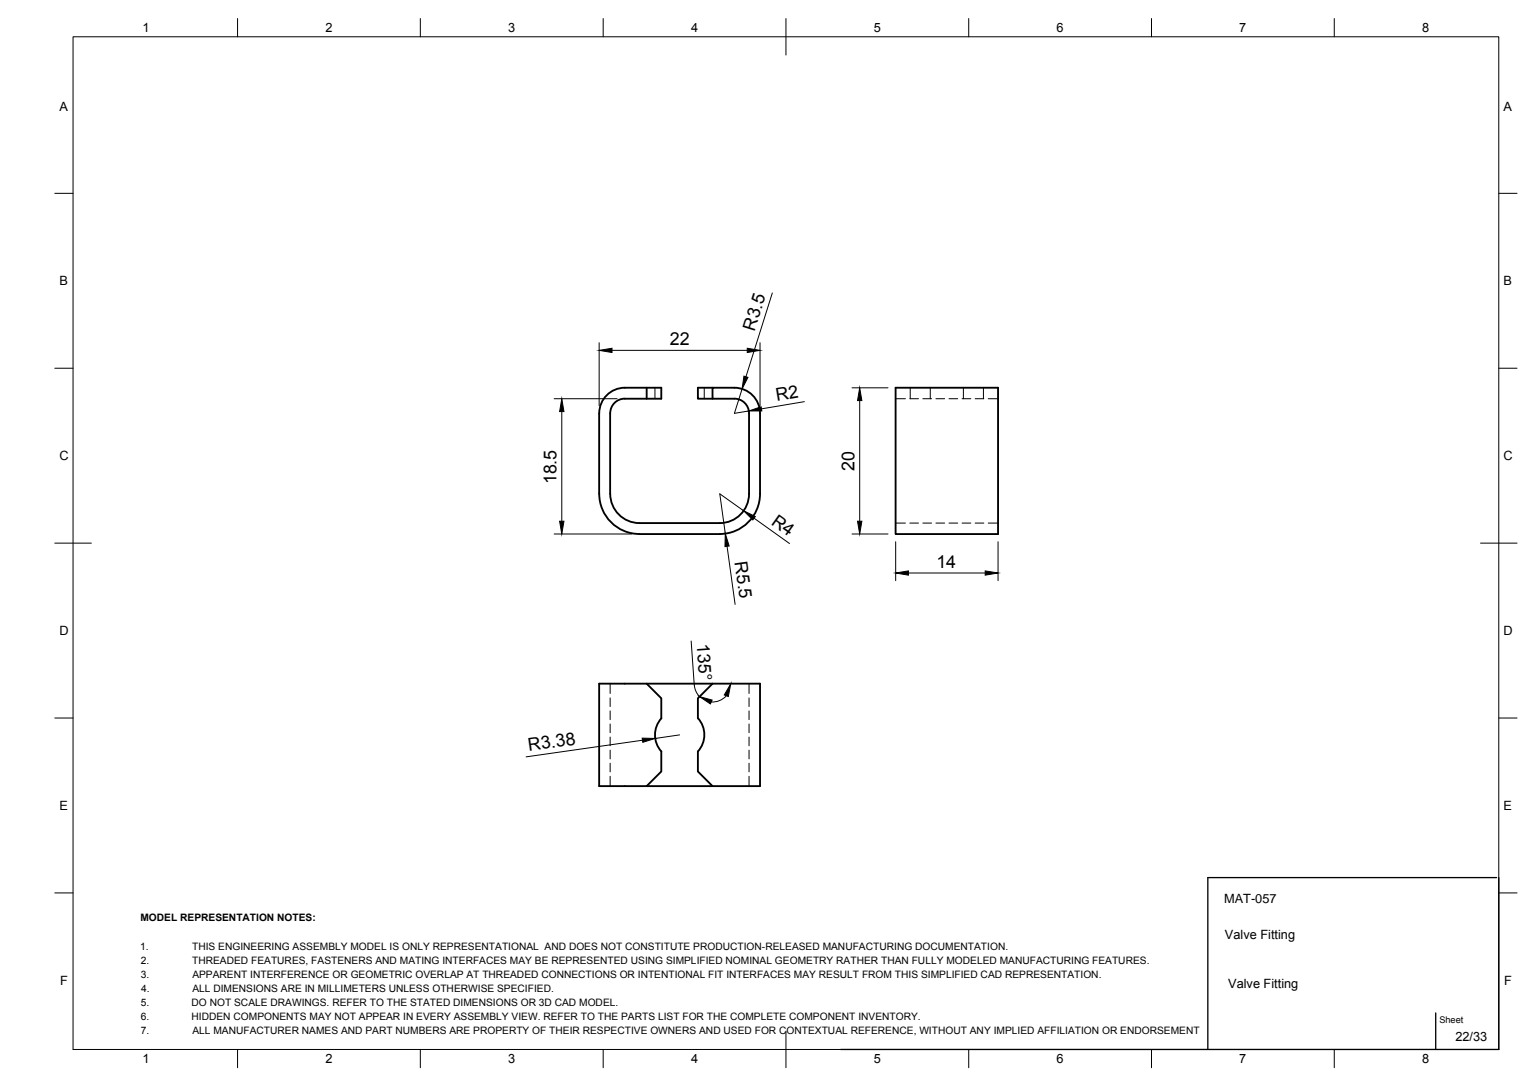
ISO-10303-21;
HEADER;
/* Generated by software containing ST-Developer
 * from STEP Tools, Inc. (www.steptools.com) 
 */

FILE_DESCRIPTION(
/* description */ ('STEP AP214', 'CAx-IF Rec.Pracs.---Representation and Presentation of Product Manufa
cturing Information (PMI)---4.0---2014-10-13'),
/* implementation_level */ '2;1');

FILE_NAME(
/* name */ 'Valve Fitting.step',
/* time_stamp */ '2026-10-28T23:34:22+01:00',
/* author */ (''),
/* organization */ (''),
/* preprocessor_version */ 'ST-DEVELOPER v20.2',
/* originating_system */ 'Autodesk Translation Framework v15.17.0.0',
/* authorisation */ '');

FILE_SCHEMA (('AP242_MANAGED_MODEL_BASED_3D_ENGINEERING_MIM_LF { 1 0 10303 442 2 1 4 }'));
ENDSEC;

DATA;
#10=MECHANICAL_DESIGN_GEOMETRIC_PRESENTATION_REPRESENTATION('',(#263),#27807);
#217=SHAPE_REPRESENTATION_RELATIONSHIP('SRR','None',#27914,#239);
#239=ADVANCED_BREP_SHAPE_REPRESENTATION('',(#292),#27794);
#263=STYLED_ITEM('',(#28070),#292);
#292=MANIFOLD_SOLID_BREP('Body1',#12039);
#645=PLANE('',#13213);
#646=PLANE('',#13215);
#647=PLANE('',#13217);
#648=PLANE('',#13226);
#649=PLANE('',#13236);
#650=PLANE('',#13238);
#651=PLANE('',#13240);
#652=PLANE('',#13242);
#653=PLANE('',#13245);
#654=PLANE('',#13247);
#655=PLANE('',#13249);
#656=PLANE('',#13251);
#657=PLANE('',#13253);
#658=PLANE('',#13255);
#659=PLANE('',#13256);
#660=PLANE('',#13258);
#661=PLANE('',#13259);
#662=PLANE('',#13260);
#663=PLANE('',#13261);
#664=PLANE('',#13262);
#1141=CYLINDRICAL_SURFACE('',#13235,3.49999999999998);
#1142=CYLINDRICAL_SURFACE('',#13237,5.50000000000002);
#1143=CYLINDRICAL_SURFACE('',#13239,5.50000000000002);
#1144=CYLINDRICAL_SURFACE('',#13241,3.49999999999998);
#1145=CYLINDRICAL_SURFACE('',#13244,1.99999999999999);
#1146=CYLINDRICAL_SURFACE('',#13246,3.99999999999998);
#1147=CYLINDRICAL_SURFACE('',#13248,3.99999999999998);
#1148=CYLINDRICAL_SURFACE('',#13250,1.99999999999999);
#1149=CYLINDRICAL_SURFACE('',#13254,3.37500000000002);
#1150=CYLINDRICAL_SURFACE('',#13257,3.37500000000002);
#1676=FACE_OUTER_BOUND('',#2452,.T.);
#1677=FACE_OUTER_BOUND('',#2453,.T.);
#1678=FACE_OUTER_BOUND('',#2454,.T.);
#1679=FACE_OUTER_BOUND('',#2455,.T.);
#1680=FACE_OUTER_BOUND('',#2456,.T.);
#1681=FACE_OUTER_BOUND('',#2457,.T.);
#1682=FACE_OUTER_BOUND('',#2458,.T.);
#1683=FACE_OUTER_BOUND('',#2459,.T.);
#1684=FACE_OUTER_BOUND('',#2460,.T.);
#1685=FACE_OUTER_BOUND('',#2461,.T.);
#1686=FACE_OUTER_BOUND('',#2462,.T.);
#1687=FACE_OUTER_BOUND('',#2463,.T.);
#1688=FACE_OUTER_BOUND('',#2464,.T.);
#1689=FACE_OUTER_BOUND('',#2465,.T.);
#1690=FACE_OUTER_BOUND('',#2466,.T.);
#1691=FACE_OUTER_BOUND('',#2467,.T.);
#1692=FACE_OUTER_BOUND('',#2468,.T.);
#1693=FACE_OUTER_BOUND('',#2469,.T.);
#1694=FACE_OUTER_BOUND('',#2470,.T.);
#1695=FACE_OUTER_BOUND('',#2471,.T.);
#1696=FACE_OUTER_BOUND('',#2472,.T.);
#1697=FACE_OUTER_BOUND('',#2473,.T.);
#1698=FACE_OUTER_BOUND('',#2474,.T.);
#1699=FACE_OUTER_BOUND('',#2475,.T.);
#1700=FACE_OUTER_BOUND('',#2476,.T.);
#1701=FACE_OUTER_BOUND('',#2477,.T.);
#1702=FACE_OUTER_BOUND('',#2478,.T.);
#1703=FACE_OUTER_BOUND('',#2479,.T.);
#1704=FACE_OUTER_BOUND('',#2480,.T.);
#1705=FACE_OUTER_BOUND('',#2481,.T.);
#2452=EDGE_LOOP('',(#9995,#9996,#9997,#9998,#9999,#10000,#10001,#10002));
#2453=EDGE_LOOP('',(#10003,#10004,#10005,#10006,#10007,#10008,#10009,#10010));
#2454=EDGE_LOOP('',(#10011,#10012,#10013,#10014,#10015,#10016,#10017,#10018,
#10019,#10020,#10021,#10022,#10023,#10024,#10025,#10026,#10027,#10028,#10029,
#10030));
#2455=EDGE_LOOP('',(#10031,#10032,#10033,#10034,#10035,#10036,#10037,#10038,
#10039,#10040,#10041,#10042,#10043,#10044,#10045,#10046,#10047,#10048,#10049,
#10050));
#2456=EDGE_LOOP('',(#10051,#10052,#10053,#10054));
#2457=EDGE_LOOP('',(#10055,#10056,#10057,#10058));
#2458=EDGE_LOOP('',(#10059,#10060,#10061,#10062));
#2459=EDGE_LOOP('',(#10063,#10064,#10065,#10066));
#2460=EDGE_LOOP('',(#10067,#10068,#10069,#10070));
#2461=EDGE_LOOP('',(#10071,#10072,#10073,#10074));
#2462=EDGE_LOOP('',(#10075,#10076,#10077,#10078));
#2463=EDGE_LOOP('',(#10079,#10080,#10081,#10082,#10083,#10084,#10085,#10086));
#2464=EDGE_LOOP('',(#10087,#10088,#10089,#10090));
#2465=EDGE_LOOP('',(#10091,#10092,#10093,#10094));
#2466=EDGE_LOOP('',(#10095,#10096,#10097,#10098));
#2467=EDGE_LOOP('',(#10099,#10100,#10101,#10102));
#2468=EDGE_LOOP('',(#10103,#10104,#10105,#10106));
#2469=EDGE_LOOP('',(#10107,#10108,#10109,#10110));
#2470=EDGE_LOOP('',(#10111,#10112,#10113,#10114));
#2471=EDGE_LOOP('',(#10115,#10116,#10117,#10118,#10119,#10120,#10121,#10122));
#2472=EDGE_LOOP('',(#10123,#10124,#10125,#10126));
#2473=EDGE_LOOP('',(#10127,#10128,#10129,#10130));
#2474=EDGE_LOOP('',(#10131,#10132,#10133,#10134));
#2475=EDGE_LOOP('',(#10135,#10136,#10137,#10138));
#2476=EDGE_LOOP('',(#10139,#10140,#10141,#10142));
#2477=EDGE_LOOP('',(#10143,#10144,#10145,#10146));
#2478=EDGE_LOOP('',(#10147,#10148,#10149,#10150));
#2479=EDGE_LOOP('',(#10151,#10152,#10153,#10154));
#2480=EDGE_LOOP('',(#10155,#10156,#10157,#10158));
#2481=EDGE_LOOP('',(#10159,#10160,#10161,#10162));
#3280=LINE('',#21304,#4100);
#3281=LINE('',#21306,#4101);
#3282=LINE('',#21308,#4102);
#3283=LINE('',#21310,#4103);
#3284=LINE('',#21312,#4104);
#3285=LINE('',#21314,#4105);
#3286=LINE('',#21316,#4106);
#3287=LINE('',#21321,#4107);
#3288=LINE('',#21323,#4108);
#3289=LINE('',#21325,#4109);
#3290=LINE('',#21329,#4110);
#3291=LINE('',#21331,#4111);
#3292=LINE('',#21333,#4112);
#3293=LINE('',#21334,#4113);
#3294=LINE('',#21336,#4114);
#3295=LINE('',#21340,#4115);
#3296=LINE('',#21344,#4116);
#3297=LINE('',#21348,#4117);
#3298=LINE('',#21352,#4118);
#3299=LINE('',#21354,#4119);
#3300=LINE('',#21356,#4120);
#3301=LINE('',#21360,#4121);
#3302=LINE('',#21364,#4122);
#3303=LINE('',#21368,#4123);
#3304=LINE('',#21373,#4124);
#3305=LINE('',#21375,#4125);
#3306=LINE('',#21377,#4126);
#3307=LINE('',#21381,#4127);
#3308=LINE('',#21385,#4128);
#3309=LINE('',#21389,#4129);
#3310=LINE('',#21391,#4130);
#3311=LINE('',#21395,#4131);
#3312=LINE('',#21399,#4132);
#3313=LINE('',#21403,#4133);
#3314=LINE('',#21406,#4134);
#3315=LINE('',#21408,#4135);
#3316=LINE('',#21410,#4136);
#3317=LINE('',#21412,#4137);
#3318=LINE('',#21414,#4138);
#3319=LINE('',#21416,#4139);
#3320=LINE('',#21418,#4140);
#3321=LINE('',#21421,#4141);
#3322=LINE('',#21423,#4142);
#3323=LINE('',#21427,#4143);
#3324=LINE('',#21428,#4144);
#3325=LINE('',#21430,#4145);
#3326=LINE('',#21432,#4146);
#3327=LINE('',#21434,#4147);
#3328=LINE('',#21436,#4148);
#3329=LINE('',#21438,#4149);
#3330=LINE('',#21440,#4150);
#3331=LINE('',#21442,#4151);
#3332=LINE('',#21446,#4152);
#3333=LINE('',#21447,#4153);
#3334=LINE('',#21449,#4154);
#3335=LINE('',#21451,#4155);
#3336=LINE('',#21454,#4156);
#3337=LINE('',#21455,#4157);
#3338=LINE('',#21457,#4158);
#3339=LINE('',#21459,#4159);
#3340=LINE('',#21461,#4160);
#3341=LINE('',#21462,#4161);
#3342=LINE('',#21464,#4162);
#3343=LINE('',#21466,#4163);
#4100=VECTOR('',#16090,1000.);
#4101=VECTOR('',#16091,1000.);
#4102=VECTOR('',#16092,1000.);
#4103=VECTOR('',#16093,1000.);
#4104=VECTOR('',#16094,1000.);
#4105=VECTOR('',#16095,1000.);
#4106=VECTOR('',#16096,1000.);
#4107=VECTOR('',#16101,1000.);
#4108=VECTOR('',#16102,1000.);
#4109=VECTOR('',#16103,1000.);
#4110=VECTOR('',#16106,1000.);
#4111=VECTOR('',#16107,1000.);
#4112=VECTOR('',#16108,1000.);
#4113=VECTOR('',#16109,1000.);
#4114=VECTOR('',#16112,1000.);
#4115=VECTOR('',#16115,1000.);
#4116=VECTOR('',#16118,1000.);
#4117=VECTOR('',#16121,1000.);
#4118=VECTOR('',#16124,1000.);
#4119=VECTOR('',#16125,1000.);
#4120=VECTOR('',#16126,1000.);
#4121=VECTOR('',#16129,1000.);
#4122=VECTOR('',#16132,1000.);
#4123=VECTOR('',#16135,1000.);
#4124=VECTOR('',#16140,1000.);
#4125=VECTOR('',#16141,1000.);
#4126=VECTOR('',#16142,1000.);
#4127=VECTOR('',#16145,1000.);
#4128=VECTOR('',#16148,1000.);
#4129=VECTOR('',#16151,1000.);
#4130=VECTOR('',#16154,1000.);
#4131=VECTOR('',#16157,1000.);
#4132=VECTOR('',#16160,1000.);
#4133=VECTOR('',#16163,1000.);
#4134=VECTOR('',#16168,1000.);
#4135=VECTOR('',#16171,1000.);
#4136=VECTOR('',#16174,1000.);
#4137=VECTOR('',#16177,1000.);
#4138=VECTOR('',#16180,1000.);
#4139=VECTOR('',#16183,1000.);
#4140=VECTOR('',#16186,1000.);
#4141=VECTOR('',#16189,1000.);
#4142=VECTOR('',#16190,1000.);
#4143=VECTOR('',#16193,1000.);
#4144=VECTOR('',#16194,1000.);
#4145=VECTOR('',#16197,1000.);
#4146=VECTOR('',#16200,1000.);
#4147=VECTOR('',#16203,1000.);
#4148=VECTOR('',#16206,1000.);
#4149=VECTOR('',#16209,1000.);
#4150=VECTOR('',#16212,1000.);
#4151=VECTOR('',#16215,1000.);
#4152=VECTOR('',#16218,1000.);
#4153=VECTOR('',#16219,1000.);
#4154=VECTOR('',#16220,1000.);
#4155=VECTOR('',#16221,1000.);
#4156=VECTOR('',#16226,1000.);
#4157=VECTOR('',#16227,1000.);
#4158=VECTOR('',#16230,1000.);
#4159=VECTOR('',#16233,1000.);
#4160=VECTOR('',#16236,1000.);
#4161=VECTOR('',#16237,1000.);
#4162=VECTOR('',#16240,1000.);
#4163=VECTOR('',#16243,1000.);
#4813=CIRCLE('',#13214,3.37500000000002);
#4814=CIRCLE('',#13216,3.37500000000002);
#4815=CIRCLE('',#13218,3.49999999999998);
#4816=CIRCLE('',#13219,5.50000000000002);
#4817=CIRCLE('',#13220,5.50000000000002);
#4818=CIRCLE('',#13221,3.49999999999998);
#4819=CIRCLE('',#13222,1.99999999999999);
#4820=CIRCLE('',#13223,3.99999999999998);
#4821=CIRCLE('',#13224,3.99999999999998);
#4822=CIRCLE('',#13225,1.99999999999999);
#4823=CIRCLE('',#13227,3.49999999999998);
#4824=CIRCLE('',#13228,5.50000000000002);
#4825=CIRCLE('',#13229,5.50000000000002);
#4826=CIRCLE('',#13230,3.49999999999998);
#4827=CIRCLE('',#13231,1.99999999999999);
#4828=CIRCLE('',#13232,3.99999999999998);
#4829=CIRCLE('',#13233,3.99999999999998);
#4830=CIRCLE('',#13234,1.99999999999999);
#4831=CIRCLE('',#13243,3.37500000000002);
#4832=CIRCLE('',#13252,3.37500000000002);
#5725=VERTEX_POINT('',#21302);
#5726=VERTEX_POINT('',#21303);
#5727=VERTEX_POINT('',#21305);
#5728=VERTEX_POINT('',#21307);
#5729=VERTEX_POINT('',#21309);
#5730=VERTEX_POINT('',#21311);
#5731=VERTEX_POINT('',#21313);
#5732=VERTEX_POINT('',#21315);
#5733=VERTEX_POINT('',#21319);
#5734=VERTEX_POINT('',#21320);
#5735=VERTEX_POINT('',#21322);
#5736=VERTEX_POINT('',#21324);
#5737=VERTEX_POINT('',#21326);
#5738=VERTEX_POINT('',#21328);
#5739=VERTEX_POINT('',#21330);
#5740=VERTEX_POINT('',#21332);
#5741=VERTEX_POINT('',#21337);
#5742=VERTEX_POINT('',#21339);
#5743=VERTEX_POINT('',#21341);
#5744=VERTEX_POINT('',#21343);
#5745=VERTEX_POINT('',#21345);
#5746=VERTEX_POINT('',#21347);
#5747=VERTEX_POINT('',#21349);
#5748=VERTEX_POINT('',#21351);
#5749=VERTEX_POINT('',#21353);
#5750=VERTEX_POINT('',#21355);
#5751=VERTEX_POINT('',#21357);
#5752=VERTEX_POINT('',#21359);
#5753=VERTEX_POINT('',#21361);
#5754=VERTEX_POINT('',#21363);
#5755=VERTEX_POINT('',#21365);
#5756=VERTEX_POINT('',#21367);
#5757=VERTEX_POINT('',#21371);
#5758=VERTEX_POINT('',#21372);
#5759=VERTEX_POINT('',#21374);
#5760=VERTEX_POINT('',#21376);
#5761=VERTEX_POINT('',#21378);
#5762=VERTEX_POINT('',#21380);
#5763=VERTEX_POINT('',#21382);
#5764=VERTEX_POINT('',#21384);
#5765=VERTEX_POINT('',#21386);
#5766=VERTEX_POINT('',#21388);
#5767=VERTEX_POINT('',#21392);
#5768=VERTEX_POINT('',#21394);
#5769=VERTEX_POINT('',#21396);
#5770=VERTEX_POINT('',#21398);
#5771=VERTEX_POINT('',#21400);
#5772=VERTEX_POINT('',#21402);
#5773=VERTEX_POINT('',#21420);
#5774=VERTEX_POINT('',#21422);
#5775=VERTEX_POINT('',#21424);
#5776=VERTEX_POINT('',#21426);
#5777=VERTEX_POINT('',#21444);
#5778=VERTEX_POINT('',#21445);
#5779=VERTEX_POINT('',#21448);
#5780=VERTEX_POINT('',#21450);
#7210=EDGE_CURVE('',#5725,#5726,#3280,.T.);
#7211=EDGE_CURVE('',#5725,#5727,#3281,.T.);
#7212=EDGE_CURVE('',#5727,#5728,#3282,.T.);
#7213=EDGE_CURVE('',#5729,#5728,#3283,.T.);
#7214=EDGE_CURVE('',#5730,#5729,#3284,.T.);
#7215=EDGE_CURVE('',#5730,#5731,#3285,.T.);
#7216=EDGE_CURVE('',#5732,#5731,#3286,.T.);
#7217=EDGE_CURVE('',#5726,#5732,#4813,.T.);
#7218=EDGE_CURVE('',#5733,#5734,#3287,.T.);
#7219=EDGE_CURVE('',#5733,#5735,#3288,.T.);
#7220=EDGE_CURVE('',#5736,#5735,#3289,.T.);
#7221=EDGE_CURVE('',#5737,#5736,#4814,.T.);
#7222=EDGE_CURVE('',#5738,#5737,#3290,.T.);
#7223=EDGE_CURVE('',#5738,#5739,#3291,.T.);
#7224=EDGE_CURVE('',#5739,#5740,#3292,.T.);
#7225=EDGE_CURVE('',#5740,#5734,#3293,.T.);
#7226=EDGE_CURVE('',#5739,#5730,#3294,.T.);
#7227=EDGE_CURVE('',#5729,#5741,#4815,.T.);
#7228=EDGE_CURVE('',#5741,#5742,#3295,.T.);
#7229=EDGE_CURVE('',#5742,#5743,#4816,.T.);
#7230=EDGE_CURVE('',#5743,#5744,#3296,.T.);
#7231=EDGE_CURVE('',#5744,#5745,#4817,.T.);
#7232=EDGE_CURVE('',#5745,#5746,#3297,.T.);
#7233=EDGE_CURVE('',#5746,#5747,#4818,.T.);
#7234=EDGE_CURVE('',#5747,#5748,#3298,.T.);
#7235=EDGE_CURVE('',#5748,#5749,#3299,.T.);
#7236=EDGE_CURVE('',#5750,#5749,#3300,.T.);
#7237=EDGE_CURVE('',#5751,#5750,#4819,.T.);
#7238=EDGE_CURVE('',#5752,#5751,#3301,.T.);
#7239=EDGE_CURVE('',#5753,#5752,#4820,.T.);
#7240=EDGE_CURVE('',#5754,#5753,#3302,.T.);
#7241=EDGE_CURVE('',#5755,#5754,#4821,.T.);
#7242=EDGE_CURVE('',#5756,#5755,#3303,.T.);
#7243=EDGE_CURVE('',#5740,#5756,#4822,.T.);
#7244=EDGE_CURVE('',#5757,#5758,#3304,.T.);
#7245=EDGE_CURVE('',#5758,#5759,#3305,.T.);
#7246=EDGE_CURVE('',#5760,#5759,#3306,.T.);
#7247=EDGE_CURVE('',#5761,#5760,#4823,.T.);
#7248=EDGE_CURVE('',#5762,#5761,#3307,.T.);
#7249=EDGE_CURVE('',#5763,#5762,#4824,.T.);
#7250=EDGE_CURVE('',#5764,#5763,#3308,.T.);
#7251=EDGE_CURVE('',#5765,#5764,#4825,.T.);
#7252=EDGE_CURVE('',#5766,#5765,#3309,.T.);
#7253=EDGE_CURVE('',#5728,#5766,#4826,.T.);
#7254=EDGE_CURVE('',#5727,#5733,#3310,.T.);
#7255=EDGE_CURVE('',#5734,#5767,#4827,.T.);
#7256=EDGE_CURVE('',#5767,#5768,#3311,.T.);
#7257=EDGE_CURVE('',#5768,#5769,#4828,.T.);
#7258=EDGE_CURVE('',#5769,#5770,#3312,.T.);
#7259=EDGE_CURVE('',#5770,#5771,#4829,.T.);
#7260=EDGE_CURVE('',#5771,#5772,#3313,.T.);
#7261=EDGE_CURVE('',#5772,#5757,#4830,.T.);
#7262=EDGE_CURVE('',#5741,#5766,#3314,.T.);
#7263=EDGE_CURVE('',#5742,#5765,#3315,.T.);
#7264=EDGE_CURVE('',#5743,#5764,#3316,.T.);
#7265=EDGE_CURVE('',#5744,#5763,#3317,.T.);
#7266=EDGE_CURVE('',#5745,#5762,#3318,.T.);
#7267=EDGE_CURVE('',#5746,#5761,#3319,.T.);
#7268=EDGE_CURVE('',#5747,#5760,#3320,.T.);
#7269=EDGE_CURVE('',#5759,#5773,#3321,.T.);
#7270=EDGE_CURVE('',#5774,#5773,#3322,.T.);
#7271=EDGE_CURVE('',#5775,#5774,#4831,.T.);
#7272=EDGE_CURVE('',#5776,#5775,#3323,.T.);
#7273=EDGE_CURVE('',#5776,#5748,#3324,.T.);
#7274=EDGE_CURVE('',#5756,#5767,#3325,.T.);
#7275=EDGE_CURVE('',#5755,#5768,#3326,.T.);
#7276=EDGE_CURVE('',#5754,#5769,#3327,.T.);
#7277=EDGE_CURVE('',#5753,#5770,#3328,.T.);
#7278=EDGE_CURVE('',#5752,#5771,#3329,.T.);
#7279=EDGE_CURVE('',#5751,#5772,#3330,.T.);
#7280=EDGE_CURVE('',#5750,#5757,#3331,.T.);
#7281=EDGE_CURVE('',#5777,#5778,#3332,.T.);
#7282=EDGE_CURVE('',#5777,#5758,#3333,.T.);
#7283=EDGE_CURVE('',#5749,#5779,#3334,.T.);
#7284=EDGE_CURVE('',#5780,#5779,#3335,.T.);
#7285=EDGE_CURVE('',#5778,#5780,#4832,.T.);
#7286=EDGE_CURVE('',#5779,#5776,#3336,.T.);
#7287=EDGE_CURVE('',#5780,#5775,#3337,.T.);
#7288=EDGE_CURVE('',#5778,#5774,#3338,.T.);
#7289=EDGE_CURVE('',#5773,#5777,#3339,.T.);
#7290=EDGE_CURVE('',#5731,#5738,#3340,.T.);
#7291=EDGE_CURVE('',#5737,#5732,#3341,.T.);
#7292=EDGE_CURVE('',#5736,#5726,#3342,.T.);
#7293=EDGE_CURVE('',#5735,#5725,#3343,.T.);
#9995=ORIENTED_EDGE('',*,*,#7210,.F.);
#9996=ORIENTED_EDGE('',*,*,#7211,.T.);
#9997=ORIENTED_EDGE('',*,*,#7212,.T.);
#9998=ORIENTED_EDGE('',*,*,#7213,.F.);
#9999=ORIENTED_EDGE('',*,*,#7214,.F.);
#10000=ORIENTED_EDGE('',*,*,#7215,.T.);
#10001=ORIENTED_EDGE('',*,*,#7216,.F.);
#10002=ORIENTED_EDGE('',*,*,#7217,.F.);
#10003=ORIENTED_EDGE('',*,*,#7218,.F.);
#10004=ORIENTED_EDGE('',*,*,#7219,.T.);
#10005=ORIENTED_EDGE('',*,*,#7220,.F.);
#10006=ORIENTED_EDGE('',*,*,#7221,.F.);
#10007=ORIENTED_EDGE('',*,*,#7222,.F.);
#10008=ORIENTED_EDGE('',*,*,#7223,.T.);
#10009=ORIENTED_EDGE('',*,*,#7224,.T.);
#10010=ORIENTED_EDGE('',*,*,#7225,.T.);
#10011=ORIENTED_EDGE('',*,*,#7224,.F.);
#10012=ORIENTED_EDGE('',*,*,#7226,.T.);
#10013=ORIENTED_EDGE('',*,*,#7214,.T.);
#10014=ORIENTED_EDGE('',*,*,#7227,.T.);
#10015=ORIENTED_EDGE('',*,*,#7228,.T.);
#10016=ORIENTED_EDGE('',*,*,#7229,.T.);
#10017=ORIENTED_EDGE('',*,*,#7230,.T.);
#10018=ORIENTED_EDGE('',*,*,#7231,.T.);
#10019=ORIENTED_EDGE('',*,*,#7232,.T.);
#10020=ORIENTED_EDGE('',*,*,#7233,.T.);
#10021=ORIENTED_EDGE('',*,*,#7234,.T.);
#10022=ORIENTED_EDGE('',*,*,#7235,.T.);
#10023=ORIENTED_EDGE('',*,*,#7236,.F.);
#10024=ORIENTED_EDGE('',*,*,#7237,.F.);
#10025=ORIENTED_EDGE('',*,*,#7238,.F.);
#10026=ORIENTED_EDGE('',*,*,#7239,.F.);
#10027=ORIENTED_EDGE('',*,*,#7240,.F.);
#10028=ORIENTED_EDGE('',*,*,#7241,.F.);
#10029=ORIENTED_EDGE('',*,*,#7242,.F.);
#10030=ORIENTED_EDGE('',*,*,#7243,.F.);
#10031=ORIENTED_EDGE('',*,*,#7244,.T.);
#10032=ORIENTED_EDGE('',*,*,#7245,.T.);
#10033=ORIENTED_EDGE('',*,*,#7246,.F.);
#10034=ORIENTED_EDGE('',*,*,#7247,.F.);
#10035=ORIENTED_EDGE('',*,*,#7248,.F.);
#10036=ORIENTED_EDGE('',*,*,#7249,.F.);
#10037=ORIENTED_EDGE('',*,*,#7250,.F.);
#10038=ORIENTED_EDGE('',*,*,#7251,.F.);
#10039=ORIENTED_EDGE('',*,*,#7252,.F.);
#10040=ORIENTED_EDGE('',*,*,#7253,.F.);
#10041=ORIENTED_EDGE('',*,*,#7212,.F.);
#10042=ORIENTED_EDGE('',*,*,#7254,.T.);
#10043=ORIENTED_EDGE('',*,*,#7218,.T.);
#10044=ORIENTED_EDGE('',*,*,#7255,.T.);
#10045=ORIENTED_EDGE('',*,*,#7256,.T.);
#10046=ORIENTED_EDGE('',*,*,#7257,.T.);
#10047=ORIENTED_EDGE('',*,*,#7258,.T.);
#10048=ORIENTED_EDGE('',*,*,#7259,.T.);
#10049=ORIENTED_EDGE('',*,*,#7260,.T.);
#10050=ORIENTED_EDGE('',*,*,#7261,.T.);
#10051=ORIENTED_EDGE('',*,*,#7253,.T.);
#10052=ORIENTED_EDGE('',*,*,#7262,.F.);
#10053=ORIENTED_EDGE('',*,*,#7227,.F.);
#10054=ORIENTED_EDGE('',*,*,#7213,.T.);
#10055=ORIENTED_EDGE('',*,*,#7252,.T.);
#10056=ORIENTED_EDGE('',*,*,#7263,.F.);
#10057=ORIENTED_EDGE('',*,*,#7228,.F.);
#10058=ORIENTED_EDGE('',*,*,#7262,.T.);
#10059=ORIENTED_EDGE('',*,*,#7251,.T.);
#10060=ORIENTED_EDGE('',*,*,#7264,.F.);
#10061=ORIENTED_EDGE('',*,*,#7229,.F.);
#10062=ORIENTED_EDGE('',*,*,#7263,.T.);
#10063=ORIENTED_EDGE('',*,*,#7250,.T.);
#10064=ORIENTED_EDGE('',*,*,#7265,.F.);
#10065=ORIENTED_EDGE('',*,*,#7230,.F.);
#10066=ORIENTED_EDGE('',*,*,#7264,.T.);
#10067=ORIENTED_EDGE('',*,*,#7249,.T.);
#10068=ORIENTED_EDGE('',*,*,#7266,.F.);
#10069=ORIENTED_EDGE('',*,*,#7231,.F.);
#10070=ORIENTED_EDGE('',*,*,#7265,.T.);
#10071=ORIENTED_EDGE('',*,*,#7248,.T.);
#10072=ORIENTED_EDGE('',*,*,#7267,.F.);
#10073=ORIENTED_EDGE('',*,*,#7232,.F.);
#10074=ORIENTED_EDGE('',*,*,#7266,.T.);
#10075=ORIENTED_EDGE('',*,*,#7247,.T.);
#10076=ORIENTED_EDGE('',*,*,#7268,.F.);
#10077=ORIENTED_EDGE('',*,*,#7233,.F.);
#10078=ORIENTED_EDGE('',*,*,#7267,.T.);
#10079=ORIENTED_EDGE('',*,*,#7246,.T.);
#10080=ORIENTED_EDGE('',*,*,#7269,.T.);
#10081=ORIENTED_EDGE('',*,*,#7270,.F.);
#10082=ORIENTED_EDGE('',*,*,#7271,.F.);
#10083=ORIENTED_EDGE('',*,*,#7272,.F.);
#10084=ORIENTED_EDGE('',*,*,#7273,.T.);
#10085=ORIENTED_EDGE('',*,*,#7234,.F.);
#10086=ORIENTED_EDGE('',*,*,#7268,.T.);
#10087=ORIENTED_EDGE('',*,*,#7255,.F.);
#10088=ORIENTED_EDGE('',*,*,#7225,.F.);
#10089=ORIENTED_EDGE('',*,*,#7243,.T.);
#10090=ORIENTED_EDGE('',*,*,#7274,.T.);
#10091=ORIENTED_EDGE('',*,*,#7256,.F.);
#10092=ORIENTED_EDGE('',*,*,#7274,.F.);
#10093=ORIENTED_EDGE('',*,*,#7242,.T.);
#10094=ORIENTED_EDGE('',*,*,#7275,.T.);
#10095=ORIENTED_EDGE('',*,*,#7257,.F.);
#10096=ORIENTED_EDGE('',*,*,#7275,.F.);
#10097=ORIENTED_EDGE('',*,*,#7241,.T.);
#10098=ORIENTED_EDGE('',*,*,#7276,.T.);
#10099=ORIENTED_EDGE('',*,*,#7258,.F.);
#10100=ORIENTED_EDGE('',*,*,#7276,.F.);
#10101=ORIENTED_EDGE('',*,*,#7240,.T.);
#10102=ORIENTED_EDGE('',*,*,#7277,.T.);
#10103=ORIENTED_EDGE('',*,*,#7259,.F.);
#10104=ORIENTED_EDGE('',*,*,#7277,.F.);
#10105=ORIENTED_EDGE('',*,*,#7239,.T.);
#10106=ORIENTED_EDGE('',*,*,#7278,.T.);
#10107=ORIENTED_EDGE('',*,*,#7260,.F.);
#10108=ORIENTED_EDGE('',*,*,#7278,.F.);
#10109=ORIENTED_EDGE('',*,*,#7238,.T.);
#10110=ORIENTED_EDGE('',*,*,#7279,.T.);
#10111=ORIENTED_EDGE('',*,*,#7261,.F.);
#10112=ORIENTED_EDGE('',*,*,#7279,.F.);
#10113=ORIENTED_EDGE('',*,*,#7237,.T.);
#10114=ORIENTED_EDGE('',*,*,#7280,.T.);
#10115=ORIENTED_EDGE('',*,*,#7281,.F.);
#10116=ORIENTED_EDGE('',*,*,#7282,.T.);
#10117=ORIENTED_EDGE('',*,*,#7244,.F.);
#10118=ORIENTED_EDGE('',*,*,#7280,.F.);
#10119=ORIENTED_EDGE('',*,*,#7236,.T.);
#10120=ORIENTED_EDGE('',*,*,#7283,.T.);
#10121=ORIENTED_EDGE('',*,*,#7284,.F.);
#10122=ORIENTED_EDGE('',*,*,#7285,.F.);
#10123=ORIENTED_EDGE('',*,*,#7284,.T.);
#10124=ORIENTED_EDGE('',*,*,#7286,.T.);
#10125=ORIENTED_EDGE('',*,*,#7272,.T.);
#10126=ORIENTED_EDGE('',*,*,#7287,.F.);
#10127=ORIENTED_EDGE('',*,*,#7285,.T.);
#10128=ORIENTED_EDGE('',*,*,#7287,.T.);
#10129=ORIENTED_EDGE('',*,*,#7271,.T.);
#10130=ORIENTED_EDGE('',*,*,#7288,.F.);
#10131=ORIENTED_EDGE('',*,*,#7270,.T.);
#10132=ORIENTED_EDGE('',*,*,#7289,.T.);
#10133=ORIENTED_EDGE('',*,*,#7281,.T.);
#10134=ORIENTED_EDGE('',*,*,#7288,.T.);
#10135=ORIENTED_EDGE('',*,*,#7216,.T.);
#10136=ORIENTED_EDGE('',*,*,#7290,.T.);
#10137=ORIENTED_EDGE('',*,*,#7222,.T.);
#10138=ORIENTED_EDGE('',*,*,#7291,.T.);
#10139=ORIENTED_EDGE('',*,*,#7221,.T.);
#10140=ORIENTED_EDGE('',*,*,#7292,.T.);
#10141=ORIENTED_EDGE('',*,*,#7217,.T.);
#10142=ORIENTED_EDGE('',*,*,#7291,.F.);
#10143=ORIENTED_EDGE('',*,*,#7220,.T.);
#10144=ORIENTED_EDGE('',*,*,#7293,.T.);
#10145=ORIENTED_EDGE('',*,*,#7210,.T.);
#10146=ORIENTED_EDGE('',*,*,#7292,.F.);
#10147=ORIENTED_EDGE('',*,*,#7282,.F.);
#10148=ORIENTED_EDGE('',*,*,#7289,.F.);
#10149=ORIENTED_EDGE('',*,*,#7269,.F.);
#10150=ORIENTED_EDGE('',*,*,#7245,.F.);
#10151=ORIENTED_EDGE('',*,*,#7219,.F.);
#10152=ORIENTED_EDGE('',*,*,#7254,.F.);
#10153=ORIENTED_EDGE('',*,*,#7211,.F.);
#10154=ORIENTED_EDGE('',*,*,#7293,.F.);
#10155=ORIENTED_EDGE('',*,*,#7223,.F.);
#10156=ORIENTED_EDGE('',*,*,#7290,.F.);
#10157=ORIENTED_EDGE('',*,*,#7215,.F.);
#10158=ORIENTED_EDGE('',*,*,#7226,.F.);
#10159=ORIENTED_EDGE('',*,*,#7283,.F.);
#10160=ORIENTED_EDGE('',*,*,#7235,.F.);
#10161=ORIENTED_EDGE('',*,*,#7273,.F.);
#10162=ORIENTED_EDGE('',*,*,#7286,.F.);
#11758=ADVANCED_FACE('',(#1676),#645,.F.);
#11759=ADVANCED_FACE('',(#1677),#646,.T.);
#11760=ADVANCED_FACE('',(#1678),#647,.T.);
#11761=ADVANCED_FACE('',(#1679),#648,.F.);
#11762=ADVANCED_FACE('',(#1680),#1141,.T.);
#11763=ADVANCED_FACE('',(#1681),#649,.F.);
#11764=ADVANCED_FACE('',(#1682),#1142,.T.);
#11765=ADVANCED_FACE('',(#1683),#650,.F.);
#11766=ADVANCED_FACE('',(#1684),#1143,.T.);
#11767=ADVANCED_FACE('',(#1685),#651,.F.);
#11768=ADVANCED_FACE('',(#1686),#1144,.T.);
#11769=ADVANCED_FACE('',(#1687),#652,.F.);
#11770=ADVANCED_FACE('',(#1688),#1145,.F.);
#11771=ADVANCED_FACE('',(#1689),#653,.T.);
#11772=ADVANCED_FACE('',(#1690),#1146,.F.);
#11773=ADVANCED_FACE('',(#1691),#654,.T.);
#11774=ADVANCED_FACE('',(#1692),#1147,.F.);
#11775=ADVANCED_FACE('',(#1693),#655,.T.);
#11776=ADVANCED_FACE('',(#1694),#1148,.F.);
#11777=ADVANCED_FACE('',(#1695),#656,.T.);
#11778=ADVANCED_FACE('',(#1696),#657,.F.);
#11779=ADVANCED_FACE('',(#1697),#1149,.F.);
#11780=ADVANCED_FACE('',(#1698),#658,.F.);
#11781=ADVANCED_FACE('',(#1699),#659,.F.);
#11782=ADVANCED_FACE('',(#1700),#1150,.F.);
#11783=ADVANCED_FACE('',(#1701),#660,.F.);
#11784=ADVANCED_FACE('',(#1702),#661,.F.);
#11785=ADVANCED_FACE('',(#1703),#662,.F.);
#11786=ADVANCED_FACE('',(#1704),#663,.T.);
#11787=ADVANCED_FACE('',(#1705),#664,.T.);
#12039=CLOSED_SHELL('',(#11758,#11759,#11760,#11761,#11762,#11763,#11764,
#11765,#11766,#11767,#11768,#11769,#11770,#11771,#11772,#11773,#11774,#11775,
#11776,#11777,#11778,#11779,#11780,#11781,#11782,#11783,#11784,#11785,#11786,
#11787));
#13212=AXIS2_PLACEMENT_3D('',#21300,#16086,#16087);
#13213=AXIS2_PLACEMENT_3D('',#21301,#16088,#16089);
#13214=AXIS2_PLACEMENT_3D('',#21317,#16097,#16098);
#13215=AXIS2_PLACEMENT_3D('',#21318,#16099,#16100);
#13216=AXIS2_PLACEMENT_3D('',#21327,#16104,#16105);
#13217=AXIS2_PLACEMENT_3D('',#21335,#16110,#16111);
#13218=AXIS2_PLACEMENT_3D('',#21338,#16113,#16114);
#13219=AXIS2_PLACEMENT_3D('',#21342,#16116,#16117);
#13220=AXIS2_PLACEMENT_3D('',#21346,#16119,#16120);
#13221=AXIS2_PLACEMENT_3D('',#21350,#16122,#16123);
#13222=AXIS2_PLACEMENT_3D('',#21358,#16127,#16128);
#13223=AXIS2_PLACEMENT_3D('',#21362,#16130,#16131);
#13224=AXIS2_PLACEMENT_3D('',#21366,#16133,#16134);
#13225=AXIS2_PLACEMENT_3D('',#21369,#16136,#16137);
#13226=AXIS2_PLACEMENT_3D('',#21370,#16138,#16139);
#13227=AXIS2_PLACEMENT_3D('',#21379,#16143,#16144);
#13228=AXIS2_PLACEMENT_3D('',#21383,#16146,#16147);
#13229=AXIS2_PLACEMENT_3D('',#21387,#16149,#16150);
#13230=AXIS2_PLACEMENT_3D('',#21390,#16152,#16153);
#13231=AXIS2_PLACEMENT_3D('',#21393,#16155,#16156);
#13232=AXIS2_PLACEMENT_3D('',#21397,#16158,#16159);
#13233=AXIS2_PLACEMENT_3D('',#21401,#16161,#16162);
#13234=AXIS2_PLACEMENT_3D('',#21404,#16164,#16165);
#13235=AXIS2_PLACEMENT_3D('',#21405,#16166,#16167);
#13236=AXIS2_PLACEMENT_3D('',#21407,#16169,#16170);
#13237=AXIS2_PLACEMENT_3D('',#21409,#16172,#16173);
#13238=AXIS2_PLACEMENT_3D('',#21411,#16175,#16176);
#13239=AXIS2_PLACEMENT_3D('',#21413,#16178,#16179);
#13240=AXIS2_PLACEMENT_3D('',#21415,#16181,#16182);
#13241=AXIS2_PLACEMENT_3D('',#21417,#16184,#16185);
#13242=AXIS2_PLACEMENT_3D('',#21419,#16187,#16188);
#13243=AXIS2_PLACEMENT_3D('',#21425,#16191,#16192);
#13244=AXIS2_PLACEMENT_3D('',#21429,#16195,#16196);
#13245=AXIS2_PLACEMENT_3D('',#21431,#16198,#16199);
#13246=AXIS2_PLACEMENT_3D('',#21433,#16201,#16202);
#13247=AXIS2_PLACEMENT_3D('',#21435,#16204,#16205);
#13248=AXIS2_PLACEMENT_3D('',#21437,#16207,#16208);
#13249=AXIS2_PLACEMENT_3D('',#21439,#16210,#16211);
#13250=AXIS2_PLACEMENT_3D('',#21441,#16213,#16214);
#13251=AXIS2_PLACEMENT_3D('',#21443,#16216,#16217);
#13252=AXIS2_PLACEMENT_3D('',#21452,#16222,#16223);
#13253=AXIS2_PLACEMENT_3D('',#21453,#16224,#16225);
#13254=AXIS2_PLACEMENT_3D('',#21456,#16228,#16229);
#13255=AXIS2_PLACEMENT_3D('',#21458,#16231,#16232);
#13256=AXIS2_PLACEMENT_3D('',#21460,#16234,#16235);
#13257=AXIS2_PLACEMENT_3D('',#21463,#16238,#16239);
#13258=AXIS2_PLACEMENT_3D('',#21465,#16241,#16242);
#13259=AXIS2_PLACEMENT_3D('',#21467,#16244,#16245);
#13260=AXIS2_PLACEMENT_3D('',#21468,#16246,#16247);
#13261=AXIS2_PLACEMENT_3D('',#21469,#16248,#16249);
#13262=AXIS2_PLACEMENT_3D('',#21470,#16250,#16251);
#16086=DIRECTION('axis',(0.,0.,1.));
#16087=DIRECTION('refdir',(1.,0.,0.));
#16088=DIRECTION('center_axis',(0.224684645967588,0.974431531646231,6.6078080723141E-17));
#16089=DIRECTION('ref_axis',(-2.99720887206891E-16,1.29778303242548E-18,
1.));
#16090=DIRECTION('',(-2.99720887206891E-16,1.29778303242547E-18,1.));
#16091=DIRECTION('',(0.689027143829045,-0.158876036792181,-0.707106781186546));
#16092=DIRECTION('',(0.974431531646231,-0.224684645967588,2.92349075108561E-16));
#16093=DIRECTION('',(2.99720887206891E-16,-1.29778303242547E-18,-1.));
#16094=DIRECTION('',(0.974431531646231,-0.224684645967588,2.92349075108561E-16));
#16095=DIRECTION('',(-0.689027143829042,0.15887603679218,-0.707106781186549));
#16096=DIRECTION('',(-2.99720887206891E-16,1.29778303242547E-18,1.));
#16097=DIRECTION('center_axis',(-0.224684645967588,-0.974431531646231,-6.6078080723141E-17));
#16098=DIRECTION('ref_axis',(1.48467301734967E-17,6.43885654072936E-17,
-1.));
#16099=DIRECTION('center_axis',(0.224684645967588,0.974431531646231,6.6078080723141E-17));
#16100=DIRECTION('ref_axis',(-2.99720887206891E-16,1.29778303242548E-18,
1.));
#16101=DIRECTION('',(0.974431531646231,-0.224684645967588,2.92349075108561E-16));
#16102=DIRECTION('',(-0.689027143829045,0.158876036792181,0.707106781186546));
#16103=DIRECTION('',(2.99720887206891E-16,-1.29778303242547E-18,-1.));
#16104=DIRECTION('center_axis',(0.224684645967588,0.974431531646231,6.6078080723141E-17));
#16105=DIRECTION('ref_axis',(-1.48467301734967E-17,-6.43885654072936E-17,
1.));
#16106=DIRECTION('',(2.99720887206891E-16,-1.29778303242547E-18,-1.));
#16107=DIRECTION('',(0.689027143829042,-0.15887603679218,0.707106781186549));
#16108=DIRECTION('',(0.974431531646231,-0.224684645967588,2.92349075108561E-16));
#16109=DIRECTION('',(2.99720887206891E-16,-1.29778303242547E-18,-1.));
#16110=DIRECTION('center_axis',(-2.99720887206891E-16,1.29778303242549E-18,
1.));
#16111=DIRECTION('ref_axis',(0.974431531646231,-0.224684645967588,2.92349075108561E-16));
#16112=DIRECTION('',(-0.224684645967588,-0.974431531646231,-6.60780807231409E-17));
#16113=DIRECTION('center_axis',(-2.99720887206891E-16,1.29778303242547E-18,
1.));
#16114=DIRECTION('ref_axis',(0.974431531646231,-0.224684645967589,2.92349075108561E-16));
#16115=DIRECTION('',(0.224684645967588,0.974431531646231,6.60780807231409E-17));
#16116=DIRECTION('center_axis',(-2.99720887206891E-16,1.29778303242547E-18,
1.));
#16117=DIRECTION('ref_axis',(0.974431531646231,-0.224684645967587,2.92349075108561E-16));
#16118=DIRECTION('',(-0.974431531646231,0.224684645967588,-2.92349075108561E-16));
#16119=DIRECTION('center_axis',(-2.99720887206891E-16,1.29778303242547E-18,
1.));
#16120=DIRECTION('ref_axis',(0.974431531646231,-0.224684645967587,2.92349075108561E-16));
#16121=DIRECTION('',(-0.224684645967588,-0.974431531646231,-6.60780807231409E-17));
#16122=DIRECTION('center_axis',(-2.99720887206891E-16,1.29778303242547E-18,
1.));
#16123=DIRECTION('ref_axis',(0.974431531646231,-0.224684645967589,2.92349075108561E-16));
#16124=DIRECTION('',(0.974431531646231,-0.224684645967588,2.92349075108561E-16));
#16125=DIRECTION('',(0.224684645967588,0.974431531646231,6.60780807231409E-17));
#16126=DIRECTION('',(0.974431531646231,-0.224684645967588,2.92349075108561E-16));
#16127=DIRECTION('center_axis',(-2.99720887206891E-16,1.29778303242547E-18,
1.));
#16128=DIRECTION('ref_axis',(-0.974431531646231,0.224684645967589,-2.92349075108561E-16));
#16129=DIRECTION('',(-0.224684645967588,-0.974431531646231,-6.60780807231409E-17));
#16130=DIRECTION('center_axis',(-2.99720887206891E-16,1.29778303242547E-18,
1.));
#16131=DIRECTION('ref_axis',(-0.974431531646231,0.224684645967589,-2.92349075108561E-16));
#16132=DIRECTION('',(-0.974431531646231,0.224684645967588,-2.92349075108561E-16));
#16133=DIRECTION('center_axis',(-2.99720887206891E-16,1.29778303242547E-18,
1.));
#16134=DIRECTION('ref_axis',(-0.974431531646231,0.224684645967589,-2.92349075108561E-16));
#16135=DIRECTION('',(0.224684645967588,0.974431531646231,6.60780807231409E-17));
#16136=DIRECTION('center_axis',(-2.99720887206891E-16,1.29778303242547E-18,
1.));
#16137=DIRECTION('ref_axis',(0.974431531646231,-0.224684645967589,2.92349075108561E-16));
#16138=DIRECTION('center_axis',(-2.99720887206891E-16,1.29778303242549E-18,
1.));
#16139=DIRECTION('ref_axis',(0.974431531646231,-0.224684645967588,2.92349075108561E-16));
#16140=DIRECTION('',(0.974431531646231,-0.224684645967588,2.92349075108561E-16));
#16141=DIRECTION('',(-0.224684645967588,-0.974431531646231,-6.60780807231409E-17));
#16142=DIRECTION('',(0.974431531646231,-0.224684645967588,2.92349075108561E-16));
#16143=DIRECTION('center_axis',(-2.99720887206891E-16,1.29778303242547E-18,
1.));
#16144=DIRECTION('ref_axis',(0.974431531646231,-0.224684645967589,2.92349075108561E-16));
#16145=DIRECTION('',(-0.224684645967588,-0.974431531646231,-6.60780807231409E-17));
#16146=DIRECTION('center_axis',(-2.99720887206891E-16,1.29778303242547E-18,
1.));
#16147=DIRECTION('ref_axis',(0.974431531646231,-0.224684645967587,2.92349075108561E-16));
#16148=DIRECTION('',(-0.974431531646231,0.224684645967588,-2.92349075108561E-16));
#16149=DIRECTION('center_axis',(-2.99720887206891E-16,1.29778303242547E-18,
1.));
#16150=DIRECTION('ref_axis',(0.974431531646231,-0.224684645967587,2.92349075108561E-16));
#16151=DIRECTION('',(0.224684645967588,0.974431531646231,6.60780807231409E-17));
#16152=DIRECTION('center_axis',(-2.99720887206891E-16,1.29778303242547E-18,
1.));
#16153=DIRECTION('ref_axis',(0.974431531646231,-0.224684645967589,2.92349075108561E-16));
#16154=DIRECTION('',(0.224684645967588,0.974431531646231,6.60780807231409E-17));
#16155=DIRECTION('center_axis',(-2.99720887206891E-16,1.29778303242547E-18,
1.));
#16156=DIRECTION('ref_axis',(0.974431531646231,-0.224684645967589,2.92349075108561E-16));
#16157=DIRECTION('',(0.224684645967588,0.974431531646231,6.60780807231409E-17));
#16158=DIRECTION('center_axis',(-2.99720887206891E-16,1.29778303242547E-18,
1.));
#16159=DIRECTION('ref_axis',(-0.974431531646231,0.224684645967589,-2.92349075108561E-16));
#16160=DIRECTION('',(-0.974431531646231,0.224684645967588,-2.92349075108561E-16));
#16161=DIRECTION('center_axis',(-2.99720887206891E-16,1.29778303242547E-18,
1.));
#16162=DIRECTION('ref_axis',(-0.974431531646231,0.224684645967589,-2.92349075108561E-16));
#16163=DIRECTION('',(-0.224684645967588,-0.974431531646231,-6.60780807231409E-17));
#16164=DIRECTION('center_axis',(-2.99720887206891E-16,1.29778303242547E-18,
1.));
#16165=DIRECTION('ref_axis',(-0.974431531646231,0.224684645967589,-2.92349075108561E-16));
#16166=DIRECTION('center_axis',(2.99720887206891E-16,-1.29778303242547E-18,
-1.));
#16167=DIRECTION('ref_axis',(-0.974431531646231,0.224684645967589,-2.92349075108561E-16));
#16168=DIRECTION('',(2.99720887206891E-16,-1.29778303242547E-18,-1.));
#16169=DIRECTION('center_axis',(-0.974431531646231,0.224684645967588,-2.92349075108561E-16));
#16170=DIRECTION('ref_axis',(-2.99720887206891E-16,1.29778303242548E-18,
1.));
#16171=DIRECTION('',(2.99720887206891E-16,-1.29778303242547E-18,-1.));
#16172=DIRECTION('center_axis',(2.99720887206891E-16,-1.29778303242547E-18,
-1.));
#16173=DIRECTION('ref_axis',(-0.974431531646231,0.224684645967587,-2.92349075108561E-16));
#16174=DIRECTION('',(2.99720887206891E-16,-1.29778303242547E-18,-1.));
#16175=DIRECTION('center_axis',(-0.224684645967588,-0.974431531646231,-6.6078080723141E-17));
#16176=DIRECTION('ref_axis',(2.99720887206891E-16,-1.29778303242548E-18,
-1.));
#16177=DIRECTION('',(2.99720887206891E-16,-1.29778303242547E-18,-1.));
#16178=DIRECTION('center_axis',(2.99720887206891E-16,-1.29778303242547E-18,
-1.));
#16179=DIRECTION('ref_axis',(-0.974431531646231,0.224684645967587,-2.92349075108561E-16));
#16180=DIRECTION('',(2.99720887206891E-16,-1.29778303242547E-18,-1.));
#16181=DIRECTION('center_axis',(0.974431531646231,-0.224684645967588,2.92349075108561E-16));
#16182=DIRECTION('ref_axis',(2.99720887206891E-16,-1.29778303242548E-18,
-1.));
#16183=DIRECTION('',(2.99720887206891E-16,-1.29778303242547E-18,-1.));
#16184=DIRECTION('center_axis',(2.99720887206891E-16,-1.29778303242547E-18,
-1.));
#16185=DIRECTION('ref_axis',(-0.974431531646231,0.224684645967589,-2.92349075108561E-16));
#16186=DIRECTION('',(2.99720887206891E-16,-1.29778303242547E-18,-1.));
#16187=DIRECTION('center_axis',(0.224684645967588,0.974431531646231,6.6078080723141E-17));
#16188=DIRECTION('ref_axis',(-2.99720887206891E-16,1.29778303242548E-18,
1.));
#16189=DIRECTION('',(0.689027143829042,-0.15887603679218,0.707106781186549));
#16190=DIRECTION('',(2.99720887206891E-16,-1.29778303242547E-18,-1.));
#16191=DIRECTION('center_axis',(-0.224684645967588,-0.974431531646231,-6.6078080723141E-17));
#16192=DIRECTION('ref_axis',(1.48467301734967E-17,6.43885654072936E-17,
-1.));
#16193=DIRECTION('',(2.99720887206891E-16,-1.29778303242547E-18,-1.));
#16194=DIRECTION('',(-0.689027143829045,0.158876036792181,0.707106781186546));
#16195=DIRECTION('center_axis',(2.99720887206891E-16,-1.29778303242547E-18,
-1.));
#16196=DIRECTION('ref_axis',(-0.974431531646231,0.224684645967589,-2.92349075108561E-16));
#16197=DIRECTION('',(2.99720887206891E-16,-1.29778303242547E-18,-1.));
#16198=DIRECTION('center_axis',(-0.974431531646231,0.224684645967588,-2.92349075108561E-16));
#16199=DIRECTION('ref_axis',(-2.99720887206891E-16,1.29778303242548E-18,
1.));
#16200=DIRECTION('',(2.99720887206891E-16,-1.29778303242547E-18,-1.));
#16201=DIRECTION('center_axis',(2.99720887206891E-16,-1.29778303242547E-18,
-1.));
#16202=DIRECTION('ref_axis',(-0.974431531646231,0.224684645967589,-2.92349075108561E-16));
#16203=DIRECTION('',(2.99720887206891E-16,-1.29778303242547E-18,-1.));
#16204=DIRECTION('center_axis',(-0.224684645967588,-0.974431531646231,-6.6078080723141E-17));
#16205=DIRECTION('ref_axis',(2.99720887206891E-16,-1.29778303242548E-18,
-1.));
#16206=DIRECTION('',(2.99720887206891E-16,-1.29778303242547E-18,-1.));
#16207=DIRECTION('center_axis',(2.99720887206891E-16,-1.29778303242547E-18,
-1.));
#16208=DIRECTION('ref_axis',(-0.974431531646231,0.224684645967589,-2.92349075108561E-16));
#16209=DIRECTION('',(2.99720887206891E-16,-1.29778303242547E-18,-1.));
#16210=DIRECTION('center_axis',(0.974431531646231,-0.224684645967588,2.92349075108561E-16));
#16211=DIRECTION('ref_axis',(2.99720887206891E-16,-1.29778303242548E-18,
-1.));
#16212=DIRECTION('',(2.99720887206891E-16,-1.29778303242547E-18,-1.));
#16213=DIRECTION('center_axis',(2.99720887206891E-16,-1.29778303242547E-18,
-1.));
#16214=DIRECTION('ref_axis',(-0.974431531646231,0.224684645967589,-2.92349075108561E-16));
#16215=DIRECTION('',(2.99720887206891E-16,-1.29778303242547E-18,-1.));
#16216=DIRECTION('center_axis',(0.224684645967588,0.974431531646231,6.6078080723141E-17));
#16217=DIRECTION('ref_axis',(-2.99720887206891E-16,1.29778303242548E-18,
1.));
#16218=DIRECTION('',(-2.99720887206891E-16,1.29778303242547E-18,1.));
#16219=DIRECTION('',(-0.689027143829042,0.15887603679218,-0.707106781186549));
#16220=DIRECTION('',(0.689027143829045,-0.158876036792181,-0.707106781186546));
#16221=DIRECTION('',(-2.99720887206891E-16,1.29778303242547E-18,1.));
#16222=DIRECTION('center_axis',(0.224684645967588,0.974431531646231,6.6078080723141E-17));
#16223=DIRECTION('ref_axis',(-1.48467301734967E-17,-6.43885654072936E-17,
1.));
#16224=DIRECTION('center_axis',(-0.974431531646231,0.224684645967588,-2.92349075108561E-16));
#16225=DIRECTION('ref_axis',(-2.99720887206891E-16,1.29778303242548E-18,
1.));
#16226=DIRECTION('',(-0.224684645967588,-0.974431531646231,-6.60780807231409E-17));
#16227=DIRECTION('',(-0.224684645967588,-0.974431531646231,-6.60780807231409E-17));
#16228=DIRECTION('center_axis',(-0.224684645967588,-0.974431531646231,-6.6078080723141E-17));
#16229=DIRECTION('ref_axis',(1.48467301734967E-17,6.43885654072935E-17,
-1.));
#16230=DIRECTION('',(-0.224684645967588,-0.974431531646231,-6.60780807231409E-17));
#16231=DIRECTION('center_axis',(-0.974431531646231,0.224684645967588,-2.92349075108561E-16));
#16232=DIRECTION('ref_axis',(-2.99720887206891E-16,1.29778303242548E-18,
1.));
#16233=DIRECTION('',(0.224684645967588,0.974431531646231,6.60780807231409E-17));
#16234=DIRECTION('center_axis',(0.974431531646231,-0.224684645967588,2.92349075108561E-16));
#16235=DIRECTION('ref_axis',(2.99720887206891E-16,-1.29778303242548E-18,
-1.));
#16236=DIRECTION('',(0.224684645967588,0.974431531646231,6.60780807231409E-17));
#16237=DIRECTION('',(-0.224684645967588,-0.974431531646231,-6.60780807231409E-17));
#16238=DIRECTION('center_axis',(-0.224684645967588,-0.974431531646231,-6.6078080723141E-17));
#16239=DIRECTION('ref_axis',(1.48467301734967E-17,6.43885654072935E-17,
-1.));
#16240=DIRECTION('',(-0.224684645967588,-0.974431531646231,-6.60780807231409E-17));
#16241=DIRECTION('center_axis',(0.974431531646231,-0.224684645967588,2.92349075108561E-16));
#16242=DIRECTION('ref_axis',(2.99720887206891E-16,-1.29778303242548E-18,
-1.));
#16243=DIRECTION('',(-0.224684645967588,-0.974431531646231,-6.60780807231409E-17));
#16244=DIRECTION('center_axis',(-0.689027143829045,0.158876036792181,0.707106781186546));
#16245=DIRECTION('ref_axis',(-0.224684645967588,-0.974431531646231,-5.55111512312579E-17));
#16246=DIRECTION('center_axis',(0.689027143829043,-0.15887603679218,0.707106781186549));
#16247=DIRECTION('ref_axis',(-0.224684645967588,-0.974431531646231,-5.55111512312579E-17));
#16248=DIRECTION('center_axis',(-0.689027143829045,0.158876036792181,0.707106781186546));
#16249=DIRECTION('ref_axis',(0.224684645967588,0.974431531646231,6.93889390390723E-17));
#16250=DIRECTION('center_axis',(0.689027143829043,-0.15887603679218,0.707106781186549));
#16251=DIRECTION('ref_axis',(0.224684645967588,0.974431531646231,5.55111512312579E-17));
#21300=CARTESIAN_POINT('',(0.,0.,0.));
#21301=CARTESIAN_POINT('Origin',(263.555188275439,150.886599378764,267.573593133704));
#21302=CARTESIAN_POINT('',(273.299503591901,148.639752919088,255.573593133704));
#21303=CARTESIAN_POINT('',(273.299503591901,148.639752919088,258.306298490302));
#21304=CARTESIAN_POINT('',(273.299503591901,148.639752919088,253.573593133704));
#21305=CARTESIAN_POINT('',(275.248366655194,148.190383627153,253.573593133704));
#21306=CARTESIAN_POINT('',(273.299503591901,148.639752919088,255.573593133704));
#21307=CARTESIAN_POINT('',(278.171661250133,147.51632968925,253.573593133704));
#21308=CARTESIAN_POINT('',(263.555188275439,150.886599378764,253.573593133704));
#21309=CARTESIAN_POINT('',(278.171661250133,147.51632968925,267.573593133704));
#21310=CARTESIAN_POINT('',(278.171661250133,147.51632968925,267.573593133704));
#21311=CARTESIAN_POINT('',(275.248366655194,148.190383627153,267.573593133704));
#21312=CARTESIAN_POINT('',(263.555188275439,150.886599378764,267.573593133704));
#21313=CARTESIAN_POINT('',(273.299503591901,148.639752919088,265.573593133704));
#21314=CARTESIAN_POINT('',(275.248366655194,148.190383627153,267.573593133704));
#21315=CARTESIAN_POINT('',(273.299503591901,148.639752919088,262.840887777106));
#21316=CARTESIAN_POINT('',(273.299503591901,148.639752919088,262.840887777106));
#21317=CARTESIAN_POINT('Origin',(270.863424762786,149.201464534007,260.573593133704));
#21318=CARTESIAN_POINT('Origin',(263.89221524439,152.348246676233,267.573593133704));
#21319=CARTESIAN_POINT('',(275.585393624145,149.652030924622,253.573593133704));
#21320=CARTESIAN_POINT('',(278.508688219084,148.97797698672,253.573593133704));
#21321=CARTESIAN_POINT('',(263.89221524439,152.348246676233,253.573593133704));
#21322=CARTESIAN_POINT('',(273.636530560853,150.101400216558,255.573593133704));
#21323=CARTESIAN_POINT('',(262.917783712744,152.572931322201,266.573593133704));
#21324=CARTESIAN_POINT('',(273.636530560853,150.101400216558,258.306298490302));
#21325=CARTESIAN_POINT('',(273.636530560853,150.101400216558,267.573593133704));
#21326=CARTESIAN_POINT('',(273.636530560853,150.101400216558,262.840887777106));
#21327=CARTESIAN_POINT('Origin',(271.200451731737,150.663111831476,260.573593133704));
#21328=CARTESIAN_POINT('',(273.636530560853,150.101400216558,265.573593133704));
#21329=CARTESIAN_POINT('',(273.636530560853,150.101400216558,267.573593133704));
#21330=CARTESIAN_POINT('',(275.585393624145,149.652030924622,267.573593133704));
#21331=CARTESIAN_POINT('',(269.738804434268,151.000138800428,261.573593133704));
#21332=CARTESIAN_POINT('',(278.508688219084,148.97797698672,267.573593133704));
#21333=CARTESIAN_POINT('',(263.89221524439,152.348246676233,267.573593133704));
#21334=CARTESIAN_POINT('',(278.508688219084,148.97797698672,267.573593133704));
#21335=CARTESIAN_POINT('Origin',(278.958057511019,150.926840050012,267.573593133704));
#21336=CARTESIAN_POINT('',(275.248366655194,148.190383627153,267.573593133704));
#21337=CARTESIAN_POINT('',(282.368567871781,150.140443789126,267.573593133704));
#21338=CARTESIAN_POINT('Origin',(278.958057511019,150.926840050012,267.573593133704));
#21339=CARTESIAN_POINT('',(284.840098977424,160.859190637234,267.573593133704));
#21340=CARTESIAN_POINT('',(282.368567871781,150.140443789126,267.573593133704));
#21341=CARTESIAN_POINT('',(280.716491106192,167.45432961411,267.573593133704));
#21342=CARTESIAN_POINT('Origin',(279.48072555337,162.094956190056,267.573593133704));
#21343=CARTESIAN_POINT('',(269.997744258083,169.925860719754,267.573593133704));
#21344=CARTESIAN_POINT('',(269.997744258083,169.925860719754,267.573593133704));
#21345=CARTESIAN_POINT('',(263.402605281207,165.802252848521,267.573593133704));
#21346=CARTESIAN_POINT('Origin',(268.761978705262,164.566487295699,267.573593133704));
#21347=CARTESIAN_POINT('',(260.931074175564,155.083506000412,267.573593133704));
#21348=CARTESIAN_POINT('',(260.931074175564,155.083506000412,267.573593133704));
#21349=CARTESIAN_POINT('',(263.555188275439,150.886599378764,267.573593133704));
#21350=CARTESIAN_POINT('Origin',(264.341584536326,154.297109739526,267.573593133704));
#21351=CARTESIAN_POINT('',(266.478482870378,150.212545440861,267.573593133704));
#21352=CARTESIAN_POINT('',(263.555188275439,150.886599378764,267.573593133704));
#21353=CARTESIAN_POINT('',(266.815509839329,151.674192738331,267.573593133704));
#21354=CARTESIAN_POINT('',(266.815509839329,151.674192738331,267.573593133704));
#21355=CARTESIAN_POINT('',(263.89221524439,152.348246676233,267.573593133704));
#21356=CARTESIAN_POINT('',(263.89221524439,152.348246676233,267.573593133704));
#21357=CARTESIAN_POINT('',(262.392721473033,154.746479031461,267.573593133704));
#21358=CARTESIAN_POINT('Origin',(264.341584536326,154.297109739526,267.573593133704));
#21359=CARTESIAN_POINT('',(264.864252578677,165.46522587957,267.573593133704));
#21360=CARTESIAN_POINT('',(262.392721473033,154.746479031461,267.573593133704));
#21361=CARTESIAN_POINT('',(269.660717289132,168.464213422284,267.573593133704));
#21362=CARTESIAN_POINT('Origin',(268.761978705262,164.566487295699,267.573593133704));
#21363=CARTESIAN_POINT('',(280.37946413724,165.992682316641,267.573593133704));
#21364=CARTESIAN_POINT('',(269.660717289132,168.464213422284,267.573593133704));
#21365=CARTESIAN_POINT('',(283.378451679955,161.196217606185,267.573593133704));
#21366=CARTESIAN_POINT('Origin',(279.48072555337,162.094956190056,267.573593133704));
#21367=CARTESIAN_POINT('',(280.906920574312,150.477470758077,267.573593133704));
#21368=CARTESIAN_POINT('',(280.906920574312,150.477470758077,267.573593133704));
#21369=CARTESIAN_POINT('Origin',(278.958057511019,150.926840050012,267.573593133704));
#21370=CARTESIAN_POINT('Origin',(278.958057511019,150.926840050012,253.573593133704));
#21371=CARTESIAN_POINT('',(263.89221524439,152.348246676233,253.573593133704));
#21372=CARTESIAN_POINT('',(266.815509839329,151.674192738331,253.573593133704));
#21373=CARTESIAN_POINT('',(263.89221524439,152.348246676233,253.573593133704));
#21374=CARTESIAN_POINT('',(266.478482870378,150.212545440861,253.573593133704));
#21375=CARTESIAN_POINT('',(267.264879131264,153.623055801623,253.573593133704));
#21376=CARTESIAN_POINT('',(263.555188275439,150.886599378764,253.573593133704));
#21377=CARTESIAN_POINT('',(263.555188275439,150.886599378764,253.573593133704));
#21378=CARTESIAN_POINT('',(260.931074175564,155.083506000412,253.573593133704));
#21379=CARTESIAN_POINT('Origin',(264.341584536326,154.297109739526,253.573593133704));
#21380=CARTESIAN_POINT('',(263.402605281207,165.802252848521,253.573593133704));
#21381=CARTESIAN_POINT('',(260.931074175564,155.083506000412,253.573593133704));
#21382=CARTESIAN_POINT('',(269.997744258083,169.925860719754,253.573593133704));
#21383=CARTESIAN_POINT('Origin',(268.761978705262,164.566487295699,253.573593133704));
#21384=CARTESIAN_POINT('',(280.716491106192,167.45432961411,253.573593133704));
#21385=CARTESIAN_POINT('',(269.997744258083,169.925860719754,253.573593133704));
#21386=CARTESIAN_POINT('',(284.840098977424,160.859190637234,253.573593133704));
#21387=CARTESIAN_POINT('Origin',(279.48072555337,162.094956190056,253.573593133704));
#21388=CARTESIAN_POINT('',(282.368567871781,150.140443789126,253.573593133704));
#21389=CARTESIAN_POINT('',(282.368567871781,150.140443789126,253.573593133704));
#21390=CARTESIAN_POINT('Origin',(278.958057511019,150.926840050012,253.573593133704));
#21391=CARTESIAN_POINT('',(276.03476291608,151.600893987915,253.573593133704));
#21392=CARTESIAN_POINT('',(280.906920574312,150.477470758077,253.573593133704));
#21393=CARTESIAN_POINT('Origin',(278.958057511019,150.926840050012,253.573593133704));
#21394=CARTESIAN_POINT('',(283.378451679955,161.196217606185,253.573593133704));
#21395=CARTESIAN_POINT('',(280.906920574312,150.477470758077,253.573593133704));
#21396=CARTESIAN_POINT('',(280.37946413724,165.992682316641,253.573593133704));
#21397=CARTESIAN_POINT('Origin',(279.48072555337,162.094956190056,253.573593133704));
#21398=CARTESIAN_POINT('',(269.660717289132,168.464213422284,253.573593133704));
#21399=CARTESIAN_POINT('',(269.660717289132,168.464213422284,253.573593133704));
#21400=CARTESIAN_POINT('',(264.864252578677,165.46522587957,253.573593133704));
#21401=CARTESIAN_POINT('Origin',(268.761978705262,164.566487295699,253.573593133704));
#21402=CARTESIAN_POINT('',(262.392721473033,154.746479031461,253.573593133704));
#21403=CARTESIAN_POINT('',(262.392721473033,154.746479031461,253.573593133704));
#21404=CARTESIAN_POINT('Origin',(264.341584536326,154.297109739526,253.573593133704));
#21405=CARTESIAN_POINT('Origin',(278.958057511019,150.926840050012,267.573593133704));
#21406=CARTESIAN_POINT('',(282.368567871781,150.140443789126,267.573593133704));
#21407=CARTESIAN_POINT('Origin',(282.368567871781,150.140443789126,267.573593133704));
#21408=CARTESIAN_POINT('',(284.840098977424,160.859190637234,267.573593133704));
#21409=CARTESIAN_POINT('Origin',(279.48072555337,162.094956190056,267.573593133704));
#21410=CARTESIAN_POINT('',(280.716491106192,167.45432961411,267.573593133704));
#21411=CARTESIAN_POINT('Origin',(269.997744258083,169.925860719754,267.573593133704));
#21412=CARTESIAN_POINT('',(269.997744258083,169.925860719754,267.573593133704));
#21413=CARTESIAN_POINT('Origin',(268.761978705262,164.566487295699,267.573593133704));
#21414=CARTESIAN_POINT('',(263.402605281207,165.802252848521,267.573593133704));
#21415=CARTESIAN_POINT('Origin',(260.931074175564,155.083506000412,267.573593133704));
#21416=CARTESIAN_POINT('',(260.931074175564,155.083506000412,267.573593133704));
#21417=CARTESIAN_POINT('Origin',(264.341584536326,154.297109739526,267.573593133704));
#21418=CARTESIAN_POINT('',(263.555188275439,150.886599378764,267.573593133704));
#21419=CARTESIAN_POINT('Origin',(263.555188275439,150.886599378764,267.573593133704));
#21420=CARTESIAN_POINT('',(268.42734593367,149.763176148926,255.573593133704));
#21421=CARTESIAN_POINT('',(266.478482870378,150.212545440861,253.573593133704));
#21422=CARTESIAN_POINT('',(268.42734593367,149.763176148926,258.306298490302));
#21423=CARTESIAN_POINT('',(268.42734593367,149.763176148926,253.573593133704));
#21424=CARTESIAN_POINT('',(268.42734593367,149.763176148926,262.840887777106));
#21425=CARTESIAN_POINT('Origin',(270.863424762786,149.201464534007,260.573593133704));
#21426=CARTESIAN_POINT('',(268.42734593367,149.763176148926,265.573593133704));
#21427=CARTESIAN_POINT('',(268.42734593367,149.763176148926,262.840887777106));
#21428=CARTESIAN_POINT('',(268.42734593367,149.763176148926,265.573593133704));
#21429=CARTESIAN_POINT('Origin',(278.958057511019,150.926840050012,267.573593133704));
#21430=CARTESIAN_POINT('',(280.906920574312,150.477470758077,267.573593133704));
#21431=CARTESIAN_POINT('Origin',(280.906920574312,150.477470758077,267.573593133704));
#21432=CARTESIAN_POINT('',(283.378451679955,161.196217606185,267.573593133704));
#21433=CARTESIAN_POINT('Origin',(279.48072555337,162.094956190056,267.573593133704));
#21434=CARTESIAN_POINT('',(280.37946413724,165.992682316641,267.573593133704));
#21435=CARTESIAN_POINT('Origin',(269.660717289132,168.464213422284,267.573593133704));
#21436=CARTESIAN_POINT('',(269.660717289132,168.464213422284,267.573593133704));
#21437=CARTESIAN_POINT('Origin',(268.761978705262,164.566487295699,267.573593133704));
#21438=CARTESIAN_POINT('',(264.864252578677,165.46522587957,267.573593133704));
#21439=CARTESIAN_POINT('Origin',(262.392721473033,154.746479031461,267.573593133704));
#21440=CARTESIAN_POINT('',(262.392721473033,154.746479031461,267.573593133704));
#21441=CARTESIAN_POINT('Origin',(264.341584536326,154.297109739526,267.573593133704));
#21442=CARTESIAN_POINT('',(263.89221524439,152.348246676233,267.573593133704));
#21443=CARTESIAN_POINT('Origin',(263.89221524439,152.348246676233,267.573593133704));
#21444=CARTESIAN_POINT('',(268.764372902622,151.224823446395,255.573593133704));
#21445=CARTESIAN_POINT('',(268.764372902622,151.224823446395,258.306298490302));
#21446=CARTESIAN_POINT('',(268.764372902622,151.224823446395,267.573593133704));
#21447=CARTESIAN_POINT('',(272.174883263383,150.438427185509,259.073593133704));
#21448=CARTESIAN_POINT('',(268.764372902622,151.224823446395,265.573593133704));
#21449=CARTESIAN_POINT('',(265.35386254186,152.011219707282,269.073593133704));
#21450=CARTESIAN_POINT('',(268.764372902622,151.224823446395,262.840887777106));
#21451=CARTESIAN_POINT('',(268.764372902622,151.224823446395,267.573593133704));
#21452=CARTESIAN_POINT('Origin',(271.200451731737,150.663111831476,260.573593133704));
#21453=CARTESIAN_POINT('Origin',(270.674192393346,159.507491465388,262.840887777106));
#21454=CARTESIAN_POINT('',(268.42734593367,149.763176148926,265.573593133704));
#21455=CARTESIAN_POINT('',(270.674192393346,159.507491465388,262.840887777106));
#21456=CARTESIAN_POINT('Origin',(273.110271222462,158.945779850469,260.573593133704));
#21457=CARTESIAN_POINT('',(270.674192393346,159.507491465388,258.306298490302));
#21458=CARTESIAN_POINT('Origin',(270.674192393346,159.507491465388,253.573593133704));
#21459=CARTESIAN_POINT('',(270.674192393346,159.507491465388,255.573593133704));
#21460=CARTESIAN_POINT('Origin',(275.546350051577,158.38406823555,262.840887777106));
#21461=CARTESIAN_POINT('',(273.636530560853,150.101400216558,265.573593133704));
#21462=CARTESIAN_POINT('',(275.546350051577,158.38406823555,262.840887777106));
#21463=CARTESIAN_POINT('Origin',(273.110271222462,158.945779850469,260.573593133704));
#21464=CARTESIAN_POINT('',(275.546350051577,158.38406823555,258.306298490302));
#21465=CARTESIAN_POINT('Origin',(275.546350051577,158.38406823555,253.573593133704));
#21466=CARTESIAN_POINT('',(275.546350051577,158.38406823555,255.573593133704));
#21467=CARTESIAN_POINT('Origin',(267.264879131264,153.623055801623,253.573593133704));
#21468=CARTESIAN_POINT('Origin',(275.546350051577,158.38406823555,255.573593133704));
#21469=CARTESIAN_POINT('Origin',(276.03476291608,151.600893987915,267.573593133704));
#21470=CARTESIAN_POINT('Origin',(270.674192393346,159.507491465388,265.573593133704));
#27765=UNCERTAINTY_MEASURE_WITH_UNIT(LENGTH_MEASURE(0.01),#27808,
'DISTANCE_ACCURACY_VALUE',
'Maximum model space distance between geometric entities at asserted c
onnectivities');
#27778=UNCERTAINTY_MEASURE_WITH_UNIT(LENGTH_MEASURE(0.01),#27808,
'DISTANCE_ACCURACY_VALUE',
'Maximum model space distance between geometric entities at asserted c
onnectivities');
#27794=(
GEOMETRIC_REPRESENTATION_CONTEXT(3)
GLOBAL_UNCERTAINTY_ASSIGNED_CONTEXT((#27765))
GLOBAL_UNIT_ASSIGNED_CONTEXT((#27808,#27810,#27811))
REPRESENTATION_CONTEXT('','3D')
);
#27807=(
GEOMETRIC_REPRESENTATION_CONTEXT(3)
GLOBAL_UNCERTAINTY_ASSIGNED_CONTEXT((#27778))
GLOBAL_UNIT_ASSIGNED_CONTEXT((#27808,#27810,#27811))
REPRESENTATION_CONTEXT('','3D')
);
#27808=(
LENGTH_UNIT()
NAMED_UNIT(*)
SI_UNIT(.MILLI.,.METRE.)
);
#27810=(
NAMED_UNIT(*)
PLANE_ANGLE_UNIT()
SI_UNIT($,.RADIAN.)
);
#27811=(
NAMED_UNIT(*)
SI_UNIT($,.STERADIAN.)
SOLID_ANGLE_UNIT()
);
#27827=SHAPE_DEFINITION_REPRESENTATION(#27860,#27914);
#27860=PRODUCT_DEFINITION_SHAPE('',$,#27943);
#27914=SHAPE_REPRESENTATION('',(#13212),#27794);
#27927=PRODUCT_DEFINITION_CONTEXT('part definition',#28013,'design');
#27943=PRODUCT_DEFINITION('Valve Fitting','Valve Fitting',#27971,#27927);
#27971=PRODUCT_DEFINITION_FORMATION('',$,#28030);
#28013=APPLICATION_CONTEXT('Managed model based 3d engineering');
#28014=PRODUCT_CONTEXT('part definition',#28013,'mechanical');
#28030=PRODUCT('Valve Fitting','Valve Fitting',$,(#28014));
#28064=COLOUR_RGB('Sky Blue',0.24,0.69,0.87);
#28065=FILL_AREA_STYLE_COLOUR('',#28064);
#28066=FILL_AREA_STYLE('',(#28065));
#28067=SURFACE_STYLE_FILL_AREA(#28066);
#28068=SURFACE_SIDE_STYLE('',(#28067));
#28069=SURFACE_STYLE_USAGE(.BOTH.,#28068);
#28070=PRESENTATION_STYLE_ASSIGNMENT((#28069));
ENDSEC;
END-ISO-10303-21;
